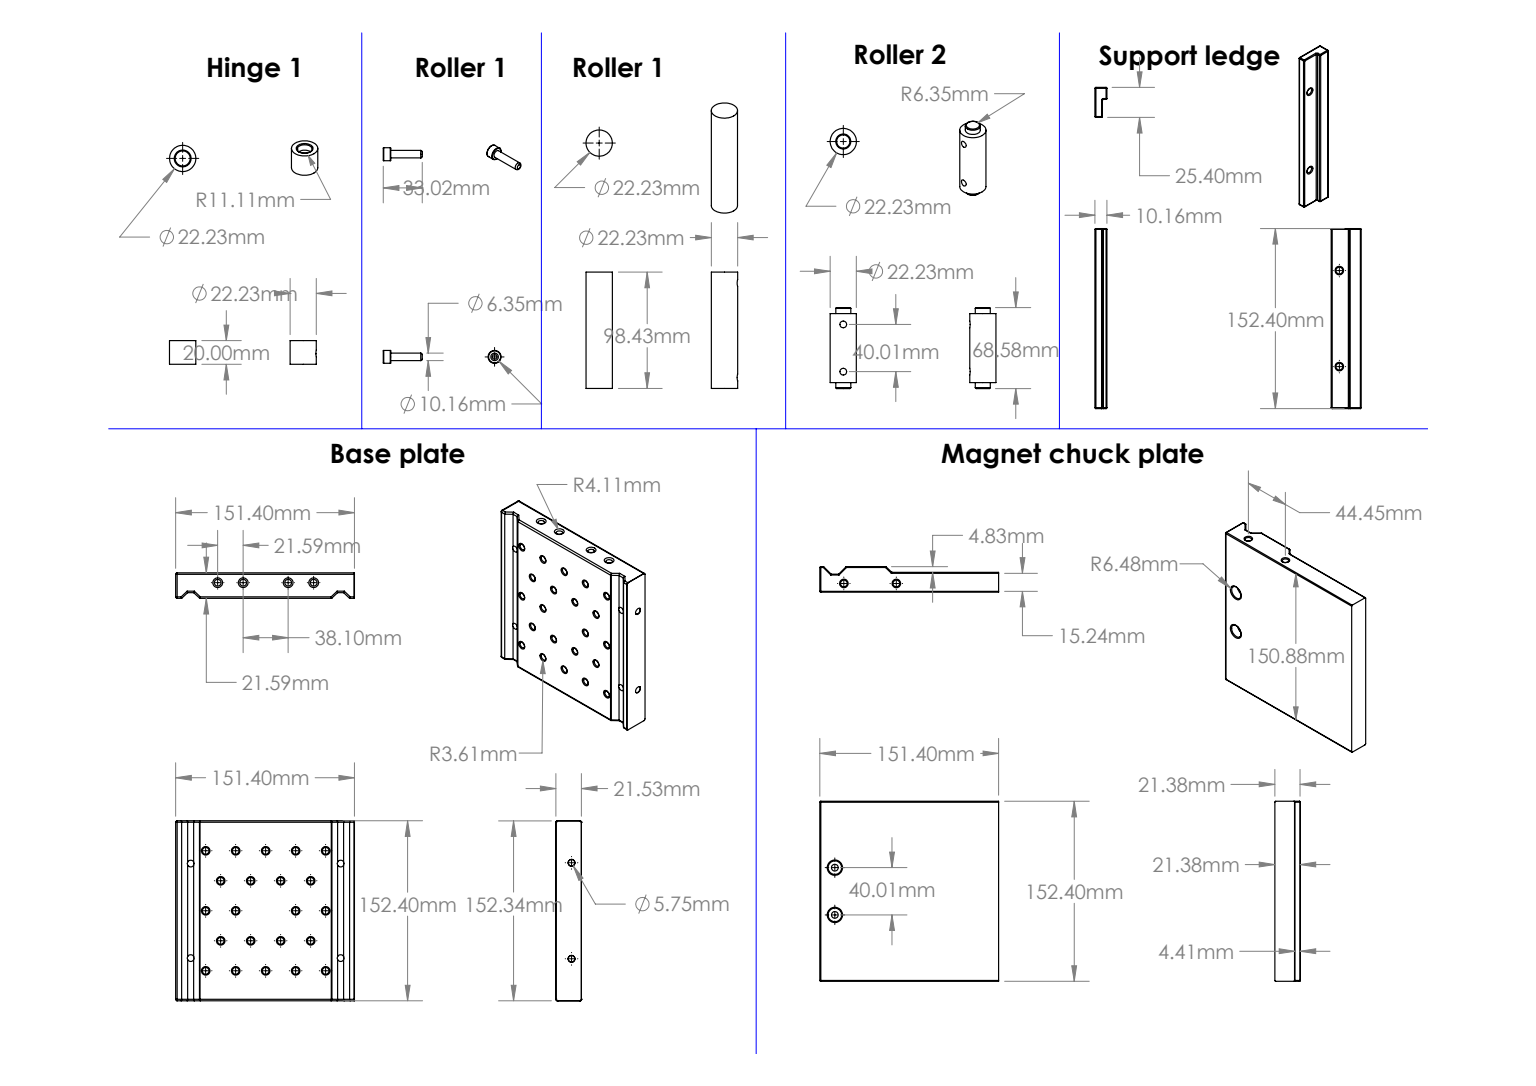
ISO-10303-21;
HEADER;
FILE_DESCRIPTION (('STEP AP214'),
    '1' );
FILE_NAME ('Hinge 1.step',
    '2026-10-26T17:37:43',
    ( '' ),
    ( '' ),
    'SwSTEP 2.0',
    'SolidWorks 2024',
    '' );
FILE_SCHEMA (( 'AUTOMOTIVE_DESIGN' ));
ENDSEC;

DATA;
#21=ORIENTED_EDGE ( 'NONE', *, *, #16592, .T. ) ;
#24=ORIENTED_EDGE ( 'NONE', *, *, #21540, .F. ) ;
#151=FACE_OUTER_BOUND ( 'NONE', #1516, .T. ) ;
#182=EDGE_CURVE ( 'NONE', #17917, #2186, #21094, .T. ) ;
#200=CIRCLE ( 'NONE', #6578, 0.7619999999999294005 ) ;
#366=CARTESIAN_POINT ( 'NONE',  ( 14.03509158661000100, -3662.022285901000032, 2257.672186979000344 ) ) ;
#368=DIRECTION ( 'NONE',  ( 0.000000000000000000, 0.000000000000000000, -1.000000000000000000 ) ) ;
#412=ORIENTED_EDGE ( 'NONE', *, *, #21540, .T. ) ;
#442=ORIENTED_EDGE ( 'NONE', *, *, #1926, .T. ) ;
#531=EDGE_CURVE ( 'NONE', #3180, #17789, #10470, .T. ) ;
#534=CARTESIAN_POINT ( 'NONE',  ( 15.54479972196000048, -3659.504990611520043, 2257.962943248000101 ) ) ;
#662=CIRCLE ( 'NONE', #16384, 11.11250000000000071 ) ;
#678=DIRECTION ( 'NONE',  ( 0.000000000000000000, 0.000000000000000000, -1.000000000000000000 ) ) ;
#714=ORIENTED_EDGE ( 'NONE', *, *, #9491, .T. ) ;
#740=EDGE_CURVE ( 'NONE', #9155, #17917, #6159, .T. ) ;
#785=PRODUCT ( 'Hinge 1', 'Hinge 1', '', ( #12191 ) ) ;
#806=ORIENTED_EDGE ( 'NONE', *, *, #17445, .T. ) ;
#1019=AXIS2_PLACEMENT_3D ( 'NONE', #14450, #2022, #21597 ) ;
#1040=ADVANCED_FACE ( 'NONE', ( #13493 ), #11393, .F. ) ;
#1091=ORIENTED_EDGE ( 'NONE', *, *, #12878, .T. ) ;
#1121=FACE_OUTER_BOUND ( 'NONE', #15842, .T. ) ;
#1168=TOROIDAL_SURFACE ( 'NONE', #14289, 7.112000000000000099, 0.7620000000000000107 ) ;
#1175=ORIENTED_EDGE ( 'NONE', *, *, #1982, .F. ) ;
#1239=AXIS2_PLACEMENT_3D ( 'NONE', #15381, #9530, #20423 ) ;
#1258=CARTESIAN_POINT ( 'NONE',  ( 12.70000020906999971, -3662.349800009999854, 2257.592639999999847 ) ) ;
#1275=PRODUCT_DEFINITION_CONTEXT ( 'detailed design', #14590, 'design' ) ;
#1366=EDGE_CURVE ( 'NONE', #17007, #3180, #17690, .T. ) ;
#1368=DIRECTION ( 'NONE',  ( 0.000000000000000000, -1.000000000000000000, 0.000000000000000000 ) ) ;
#1370=ORIENTED_EDGE ( 'NONE', *, *, #16592, .F. ) ;
#1382=CARTESIAN_POINT ( 'NONE',  ( 12.42421805959000025, -3662.340875907999816, 2257.594929573999707 ) ) ;
#1445=ORIENTED_EDGE ( 'NONE', *, *, #1366, .F. ) ;
#1489=CARTESIAN_POINT ( 'NONE',  ( 9.970475488813999476, -3658.687501247999990, 2257.932973791000222 ) ) ;
#1490=CARTESIAN_POINT ( 'NONE',  ( 11.12257588577000078, -3661.878010978000020, 2257.704312134999782 ) ) ;
#1516=EDGE_LOOP ( 'NONE', ( #13022, #20332, #9666, #3962 ) ) ;
#1545=AXIS2_PLACEMENT_3D ( 'NONE', #16930, #6293, #20459 ) ;
#1549=AXIS2_PLACEMENT_3D ( 'NONE', #16667, #9524, #18765 ) ;
#1593=VERTEX_POINT ( 'NONE', #21921 ) ;
#1607=CARTESIAN_POINT ( 'NONE',  ( 9.855200508358999301, -3659.413078923999819, 2257.962940201000038 ) ) ;
#1611=CARTESIAN_POINT ( 'NONE',  ( 12.69999999999999929, -3649.471999999999753, 2262.355140000000119 ) ) ;
#1732=CARTESIAN_POINT ( 'NONE',  ( 12.69999999999999929, -3655.060000000000400, 2268.705139999999574 ) ) ;
#1803=EDGE_LOOP ( 'NONE', ( #3126, #6623 ) ) ;
#1851=CARTESIAN_POINT ( 'NONE',  ( 10.49453184711000020, -3657.700682589000280, 2257.813182895999944 ) ) ;
#1876=DIRECTION ( 'NONE',  ( 0.000000000000000000, -1.000000000000000000, 0.000000000000000000 ) ) ;
#1926=EDGE_CURVE ( 'NONE', #5052, #15577, #13332, .T. ) ;
#1982=EDGE_CURVE ( 'NONE', #2186, #17917, #3455, .T. ) ;
#1998=DIRECTION ( 'NONE',  ( 0.000000000000000000, 0.000000000000000000, 1.000000000000000000 ) ) ;
#2016=PLANE ( 'NONE',  #20971 ) ;
#2022=DIRECTION ( 'NONE',  ( 0.000000000000000000, 1.000000000000000000, 0.000000000000000000 ) ) ;
#2056=VECTOR ( 'NONE', #21267, 1000.000000000000000 ) ;
#2132=CARTESIAN_POINT ( 'NONE',  ( 15.42948858069999929, -3660.322618741000042, 2257.932964559000084 ) ) ;
#2179=ORIENTED_EDGE ( 'NONE', *, *, #9491, .F. ) ;
#2186=VERTEX_POINT ( 'NONE', #13680 ) ;
#2241=ORIENTED_EDGE ( 'NONE', *, *, #182, .T. ) ;
#2257=( GEOMETRIC_REPRESENTATION_CONTEXT ( 3 ) GLOBAL_UNCERTAINTY_ASSIGNED_CONTEXT ( ( #16741 ) ) GLOBAL_UNIT_ASSIGNED_CONTEXT ( ( #21126, #3419, #23094 ) ) REPRESENTATION_CONTEXT ( 'NONE', 'WORKASPACE' ) );
#2282=DIRECTION ( 'NONE',  ( -1.000000000000000000, -0.000000000000000000, -0.000000000000000000 ) ) ;
#2451=CARTESIAN_POINT ( 'NONE',  ( 12.69999999999999929, -3655.060000000000400, 2262.355140000000119 ) ) ;
#2490=LINE ( 'NONE', #22263, #21072 ) ;
#2547=AXIS2_PLACEMENT_3D ( 'NONE', #19457, #3285, #21103 ) ;
#2606=CARTESIAN_POINT ( 'NONE',  ( 0.000000000000000000, 0.000000000000000000, 0.000000000000000000 ) ) ;
#2739=CARTESIAN_POINT ( 'NONE',  ( 12.69999999999999929, -3655.060000000000400, 2262.355140000000119 ) ) ;
#2769=DIRECTION ( 'NONE',  ( 0.000000000000000000, -1.000000000000000000, 0.000000000000000000 ) ) ;
#2788=CARTESIAN_POINT ( 'NONE',  ( 12.69999999999999929, -3656.660200000000259, 2257.592639999999847 ) ) ;
#2865=DIRECTION ( 'NONE',  ( 1.000000000000000000, 0.000000000000000000, 0.000000000000000000 ) ) ;
#2910=CARTESIAN_POINT ( 'NONE',  ( 9.855200508393229697, -3659.504999998446692, 2257.962940200992307 ) ) ;
#3080=ORIENTED_EDGE ( 'NONE', *, *, #3865, .F. ) ;
#3126=ORIENTED_EDGE ( 'NONE', *, *, #15553, .T. ) ;
#3140=CARTESIAN_POINT ( 'NONE',  ( 14.03517516284999900, -3656.987758144000054, 2257.672197071000028 ) ) ;
#3156=EDGE_LOOP ( 'NONE', ( #12594, #412 ) ) ;
#3180=VERTEX_POINT ( 'NONE', #6414 ) ;
#3206=CIRCLE ( 'NONE', #5096, 11.11250000000000071 ) ;
#3208=LINE ( 'NONE', #13881, #2056 ) ;
#3257=CARTESIAN_POINT ( 'NONE',  ( 12.15081356636999921, -3656.709137308999743, 2257.605105499000274 ) ) ;
#3258=CARTESIAN_POINT ( 'NONE',  ( 9.855200958505918152, -3659.596994900638038, 2257.962940081783472 ) ) ;
#3285=DIRECTION ( 'NONE',  ( 0.000000000000000000, -1.000000000000000000, 0.000000000000000000 ) ) ;
#3316=VERTEX_POINT ( 'NONE', #3346 ) ;
#3346=CARTESIAN_POINT ( 'NONE',  ( 12.69999999999999929, -3655.060000000000400, 2275.055139999999483 ) ) ;
#3419=( NAMED_UNIT ( * ) PLANE_ANGLE_UNIT ( ) SI_UNIT ( $, .RADIAN. ) );
#3450=AXIS2_PLACEMENT_3D ( 'NONE', #4410, #9682, #6296 ) ;
#3455=CIRCLE ( 'NONE', #8332, 6.349999999999855760 ) ;
#3630=CARTESIAN_POINT ( 'NONE',  ( 12.69999999999999929, -3648.710000000000036, 2268.705139999999574 ) ) ;
#3646=CARTESIAN_POINT ( 'NONE',  ( 12.79204376678999999, -3662.349799990000065, 2257.592639999999847 ) ) ;
#3651=CARTESIAN_POINT ( 'NONE',  ( 12.69999999999999929, -3655.060000000000400, 2268.705139999999574 ) ) ;
#3691=ADVANCED_FACE ( 'NONE', ( #151 ), #7297, .F. ) ;
#3753=DIRECTION ( 'NONE',  ( 1.000000000000000000, 0.000000000000000000, -1.224646799147353207E-16 ) ) ;
#3815=DIRECTION ( 'NONE',  ( 0.000000000000000000, 0.000000000000000000, -1.000000000000000000 ) ) ;
#3865=EDGE_CURVE ( 'NONE', #3889, #15577, #4425, .T. ) ;
#3889=VERTEX_POINT ( 'NONE', #14792 ) ;
#3962=ORIENTED_EDGE ( 'NONE', *, *, #182, .F. ) ;
#4078=ORIENTED_EDGE ( 'NONE', *, *, #13162, .T. ) ;
#4242=CIRCLE ( 'NONE', #4993, 7.111999999999785160 ) ;
#4284=CARTESIAN_POINT ( 'NONE',  ( 12.69999999999999929, -3648.710000000000036, 2268.705139999999574 ) ) ;
#4338=TOROIDAL_SURFACE ( 'NONE', #11437, 7.112000000000000099, 0.7620000000000000107 ) ;
#4410=CARTESIAN_POINT ( 'NONE',  ( 12.69999999999999929, -3659.504999999999654, 2272.030000000000200 ) ) ;
#4425=B_SPLINE_CURVE_WITH_KNOTS ( 'NONE', 3,
 ( #5899, #13036, #11267, #18414 ),
 .UNSPECIFIED., .F., .F.,
 ( 4, 4 ),
 ( 0.000000000000000000, 3.168591426078622932E-06 ),
 .UNSPECIFIED. ) ;
#4428=DIRECTION ( 'NONE',  ( 0.000000000000000000, -1.000000000000000000, 0.000000000000000000 ) ) ;
#4511=EDGE_CURVE ( 'NONE', #8413, #3889, #6339, .T. ) ;
#4544=CARTESIAN_POINT ( 'NONE',  ( 14.27729191008000065, -3657.131900051000230, 2257.704292951999832 ) ) ;
#4585=CIRCLE ( 'NONE', #14342, 11.11250000000000071 ) ;
#4649=CIRCLE ( 'NONE', #13636, 2.844799999999999773 ) ;
#4722=CARTESIAN_POINT ( 'NONE',  ( 12.70000000000000107, -3668.712499999999636, 2279.817639999999756 ) ) ;
#4746=CARTESIAN_POINT ( 'NONE',  ( 12.69999999999999929, -3668.712499999999636, 2268.705139999999574 ) ) ;
#4883=LINE ( 'NONE', #17411, #16568 ) ;
#4898=CARTESIAN_POINT ( 'NONE',  ( 10.32639513556999944, -3661.081539619000068, 2257.848705702999723 ) ) ;
#4936=DIRECTION ( 'NONE',  ( 0.000000000000000000, -1.000000000000000000, 0.000000000000000000 ) ) ;
#4993=AXIS2_PLACEMENT_3D ( 'NONE', #3630, #1876, #1998 ) ;
#5021=CARTESIAN_POINT ( 'NONE',  ( 9.855200508358999301, -3659.504986005999854, 2257.962940201000038 ) ) ;
#5032=ORIENTED_EDGE ( 'NONE', *, *, #12878, .F. ) ;
#5052=VERTEX_POINT ( 'NONE', #22901 ) ;
#5096=AXIS2_PLACEMENT_3D ( 'NONE', #8757, #14264, #10622 ) ;
#5144=CARTESIAN_POINT ( 'NONE',  ( 10.18227454630999951, -3660.839269783999953, 2257.881334183000035 ) ) ;
#5186=VERTEX_POINT ( 'NONE', #16684 ) ;
#5254=CARTESIAN_POINT ( 'NONE',  ( 12.69999999999999929, -3659.504999999999654, 2272.030000000000200 ) ) ;
#5439=EDGE_LOOP ( 'NONE', ( #1091, #9150 ) ) ;
#5541=CARTESIAN_POINT ( 'NONE',  ( 15.21766708706000060, -3660.839381832000072, 2257.881320499000140 ) ) ;
#5605=DIRECTION ( 'NONE',  ( 0.000000000000000000, 0.000000000000000000, -1.000000000000000000 ) ) ;
#5611=AXIS2_PLACEMENT_3D ( 'NONE', #2606, #9751, #7545 ) ;
#5680=CIRCLE ( 'NONE', #7178, 6.349999999999855760 ) ;
#5770=CARTESIAN_POINT ( 'NONE',  ( 13.24911585008999815, -3662.300876935000360, 2257.605101898000157 ) ) ;
#5801=( LENGTH_UNIT ( ) NAMED_UNIT ( * ) SI_UNIT ( .MILLI., .METRE. ) );
#5815=EDGE_CURVE ( 'NONE', #17789, #8413, #6051, .T. ) ;
#5838=MANIFOLD_SOLID_BREP ( 'SOLID2-15[1]', #16587 ) ;
#5899=CARTESIAN_POINT ( 'NONE',  ( 9.855200508358999301, -3659.504986005999854, 2257.962940201000038 ) ) ;
#5928=ORIENTED_EDGE ( 'NONE', *, *, #13887, .F. ) ;
#5991=EDGE_CURVE ( 'NONE', #6867, #3180, #10524, .T. ) ;
#6027=( NAMED_UNIT ( * ) PLANE_ANGLE_UNIT ( ) SI_UNIT ( $, .RADIAN. ) );
#6028=FACE_OUTER_BOUND ( 'NONE', #11655, .T. ) ;
#6051=B_SPLINE_CURVE_WITH_KNOTS ( 'NONE', 3,
 ( #6557, #10051, #12047, #17081, #6678, #11814, #19203, #6786, #13816, #13927, #13457, #4544, #3140, #22584, #11687, #18844, #21077, #8074, #2788 ),
 .UNSPECIFIED., .F., .F.,
 ( 4, 1, 1, 1, 1, 1, 1, 1, 1, 1, 1, 1, 1, 1, 1, 1, 4 ),
 ( 0.000000000000000000, 0.06250000000000000000, 0.1250000000000000000, 0.1875000000000000000, 0.2500000000000000000, 0.3125000000000000000, 0.3750000000000000000, 0.4375000000000000000, 0.5000000000000000000, 0.5625000000000000000, 0.6250000000000000000, 0.6875000000000000000, 0.7500000000000000000, 0.8125000000000000000, 0.8750000000000000000, 0.9375000000000000000, 1.000000000000000000 ),
 .UNSPECIFIED. ) ;
#6159=LINE ( 'NONE', #2739, #19136 ) ;
#6179=ORIENTED_EDGE ( 'NONE', *, *, #13727, .T. ) ;
#6188=DIRECTION ( 'NONE',  ( 0.000000000000000000, 0.000000000000000000, -1.000000000000000000 ) ) ;
#6293=DIRECTION ( 'NONE',  ( 0.000000000000000000, 1.000000000000000000, 0.000000000000000000 ) ) ;
#6296=DIRECTION ( 'NONE',  ( -1.000000000000000000, 0.000000000000000000, 0.000000000000000000 ) ) ;
#6339=B_SPLINE_CURVE_WITH_KNOTS ( 'NONE', 3,
 ( #21423, #7025, #12164, #3257, #21542, #13924, #10403, #17543, #19785, #19544, #1851, #6784, #22925, #19430, #1489, #10632, #14393, #1607, #5021 ),
 .UNSPECIFIED., .F., .F.,
 ( 4, 1, 1, 1, 1, 1, 1, 1, 1, 1, 1, 1, 1, 1, 1, 1, 4 ),
 ( 0.000000000000000000, 0.06250000000000000000, 0.1250000000000000000, 0.1875000000000000000, 0.2500000000000000000, 0.3125000000000000000, 0.3750000000000000000, 0.4375000000000000000, 0.5000000000000000000, 0.5625000000000000000, 0.6250000000000000000, 0.6875000000000000000, 0.7500000000000000000, 0.8125000000000000000, 0.8750000000000000000, 0.9375000000000000000, 1.000000000000000000 ),
 .UNSPECIFIED. ) ;
#6414=CARTESIAN_POINT ( 'NONE',  ( 15.54479972192533488, -3659.504999998566745, 2257.962943247991007 ) ) ;
#6557=CARTESIAN_POINT ( 'NONE',  ( 15.54479972196000048, -3659.504985917999875, 2257.962943248000101 ) ) ;
#6578=AXIS2_PLACEMENT_3D ( 'NONE', #19825, #3753, #368 ) ;
#6608=CARTESIAN_POINT ( 'NONE',  ( 12.69999999999999929, -3648.710000000000036, 2268.705139999999574 ) ) ;
#6623=ORIENTED_EDGE ( 'NONE', *, *, #15321, .T. ) ;
#6676=CARTESIAN_POINT ( 'NONE',  ( 9.864080040025308804, -3659.780148078739330, 2257.960588549625299 ) ) ;
#6678=CARTESIAN_POINT ( 'NONE',  ( 15.42952381853999988, -3658.687498958000106, 2257.932973515999947 ) ) ;
#6721=CARTESIAN_POINT ( 'NONE',  ( 12.69999999999999929, -3648.710000000000036, 2257.592639999999847 ) ) ;
#6753=DIRECTION ( 'NONE',  ( 0.000000000000000000, -1.000000000000000000, 0.000000000000000000 ) ) ;
#6784=CARTESIAN_POINT ( 'NONE',  ( 10.32641459757000035, -3657.928429337000125, 2257.848701351999807 ) ) ;
#6786=CARTESIAN_POINT ( 'NONE',  ( 15.07358448401000217, -3657.928427944000305, 2257.848701151000114 ) ) ;
#6867=VERTEX_POINT ( 'NONE', #20304 ) ;
#6920=FACE_OUTER_BOUND ( 'NONE', #3156, .T. ) ;
#6934=CARTESIAN_POINT ( 'NONE',  ( 12.69999999999999929, -3648.710000000000036, 2261.593139999999948 ) ) ;
#6985=SHAPE_REPRESENTATION ( 'Hinge 1', ( #5611 ), #14218 ) ;
#7025=CARTESIAN_POINT ( 'NONE',  ( 12.60791899384999937, -3656.660200000000259, 2257.592639999999847 ) ) ;
#7027=VERTEX_POINT ( 'NONE', #6934 ) ;
#7038=VECTOR ( 'NONE', #16603, 1000.000000000000000 ) ;
#7178=AXIS2_PLACEMENT_3D ( 'NONE', #1732, #16253, #5605 ) ;
#7245=DIRECTION ( 'NONE',  ( 0.000000000000000000, -1.000000000000000000, 0.000000000000000000 ) ) ;
#7297=CYLINDRICAL_SURFACE ( 'NONE', #1019, 6.349999999999855760 ) ;
#7358=AXIS2_PLACEMENT_3D ( 'NONE', #4284, #18576, #7914 ) ;
#7425=VERTEX_POINT ( 'NONE', #4722 ) ;
#7459=ADVANCED_FACE ( 'NONE', ( #10098 ), #12330, .T. ) ;
#7510=CARTESIAN_POINT ( 'NONE',  ( 15.49598722424000030, -3660.053501552999933, 2257.950090894999903 ) ) ;
#7540=CIRCLE ( 'NONE', #1545, 6.349999999999855760 ) ;
#7545=DIRECTION ( 'NONE',  ( 1.000000000000000000, 0.000000000000000000, 0.000000000000000000 ) ) ;
#7637=ADVANCED_FACE ( 'NONE', ( #16418 ), #2016, .T. ) ;
#7677=CARTESIAN_POINT ( 'NONE',  ( 15.54479972196000048, -3659.504985917999875, 2257.962943248000101 ) ) ;
#7732=SHAPE_DEFINITION_REPRESENTATION ( #20441, #6985 ) ;
#7837=UNCERTAINTY_MEASURE_WITH_UNIT (LENGTH_MEASURE( 1.000000000000000082E-05 ), #5801, 'distance_accuracy_value', 'NONE');
#7914=DIRECTION ( 'NONE',  ( 0.000000000000000000, 0.000000000000000000, 1.000000000000000000 ) ) ;
#7943=CARTESIAN_POINT ( 'NONE',  ( 12.69999999999999929, -3648.710000000000036, 2268.705139999999574 ) ) ;
#7944=CIRCLE ( 'NONE', #21045, 11.11250000000000071 ) ;
#7948=CARTESIAN_POINT ( 'NONE',  ( 9.855199999999999960, -3659.504999999999654, 2272.030000000000200 ) ) ;
#8065=FACE_OUTER_BOUND ( 'NONE', #11000, .T. ) ;
#8074=CARTESIAN_POINT ( 'NONE',  ( 12.79208108087000006, -3656.660200000000259, 2257.592639999999847 ) ) ;
#8172=CARTESIAN_POINT ( 'NONE',  ( 12.69999999999999929, -3649.471999999999753, 2268.705139999999574 ) ) ;
#8180=DIRECTION ( 'NONE',  ( -1.000000000000000000, 0.000000000000000000, 0.000000000000000000 ) ) ;
#8223=CARTESIAN_POINT ( 'NONE',  ( 12.69999999999999929, -3649.471999999999753, 2268.705139999999574 ) ) ;
#8231=ORIENTED_EDGE ( 'NONE', *, *, #1926, .F. ) ;
#8248=PRODUCT_DEFINITION_FORMATION_WITH_SPECIFIED_SOURCE ( 'ANY', '', #785, .NOT_KNOWN. ) ;
#8305=CARTESIAN_POINT ( 'NONE',  ( 11.61844525849999954, -3662.141125287999785, 2257.644379465999918 ) ) ;
#8309=ORIENTED_EDGE ( 'NONE', *, *, #10357, .F. ) ;
#8332=AXIS2_PLACEMENT_3D ( 'NONE', #20479, #4428, #18374 ) ;
#8413=VERTEX_POINT ( 'NONE', #13272 ) ;
#8462=CIRCLE ( 'NONE', #13691, 2.844799999999999773 ) ;
#8560=VERTEX_POINT ( 'NONE', #6721 ) ;
#8757=CARTESIAN_POINT ( 'NONE',  ( 12.69999999999999929, -3668.712499999999636, 2268.705139999999574 ) ) ;
#8831=ORIENTED_EDGE ( 'NONE', *, *, #5991, .T. ) ;
#8888=DIRECTION ( 'NONE',  ( 1.000000000000000000, 0.000000000000000000, 0.000000000000000000 ) ) ;
#8955=ADVANCED_FACE ( 'NONE', ( #6920 ), #13834, .T. ) ;
#9150=ORIENTED_EDGE ( 'NONE', *, *, #10357, .T. ) ;
#9155=VERTEX_POINT ( 'NONE', #2451 ) ;
#9188=ORIENTED_EDGE ( 'NONE', *, *, #5815, .F. ) ;
#9318=CARTESIAN_POINT ( 'NONE',  ( 12.69999999999999929, -3649.471999999999753, 2261.593139999999948 ) ) ;
#9491=EDGE_CURVE ( 'NONE', #8560, #1593, #662, .T. ) ;
#9524=DIRECTION ( 'NONE',  ( 0.000000000000000000, 0.000000000000000000, 1.000000000000000000 ) ) ;
#9530=DIRECTION ( 'NONE',  ( 0.000000000000000000, 1.000000000000000000, 0.000000000000000000 ) ) ;
#9559=DIRECTION ( 'NONE',  ( 0.000000000000000000, -1.000000000000000000, 0.000000000000000000 ) ) ;
#9666=ORIENTED_EDGE ( 'NONE', *, *, #17249, .T. ) ;
#9682=DIRECTION ( 'NONE',  ( 0.000000000000000000, 0.000000000000000000, -1.000000000000000000 ) ) ;
#9751=DIRECTION ( 'NONE',  ( 0.000000000000000000, 0.000000000000000000, 1.000000000000000000 ) ) ;
#9857=ORIENTED_EDGE ( 'NONE', *, *, #17445, .F. ) ;
#9865=ORIENTED_EDGE ( 'NONE', *, *, #16471, .T. ) ;
#9923=ADVANCED_FACE ( 'NONE', ( #16878, #11494 ), #18644, .F. ) ;
#10049=CARTESIAN_POINT ( 'NONE',  ( 9.904004635912999177, -3660.053455317999578, 2257.950092655999924 ) ) ;
#10051=CARTESIAN_POINT ( 'NONE',  ( 15.54479972196000048, -3659.413078500999745, 2257.962943248000101 ) ) ;
#10098=FACE_OUTER_BOUND ( 'NONE', #18381, .T. ) ;
#10239=EDGE_CURVE ( 'NONE', #15577, #17007, #22466, .T. ) ;
#10285=CARTESIAN_POINT ( 'NONE',  ( 9.970491213060000746, -3660.322548418000224, 2257.932969814999979 ) ) ;
#10357=EDGE_CURVE ( 'NONE', #6867, #5052, #8462, .T. ) ;
#10403=CARTESIAN_POINT ( 'NONE',  ( 11.36482343738000012, -3656.987758866999684, 2257.672197237000091 ) ) ;
#10470=B_SPLINE_CURVE_WITH_KNOTS ( 'NONE', 3,
 ( #21639, #16581, #534, #7677 ),
 .UNSPECIFIED., .F., .F.,
 ( 4, 4 ),
 ( 0.9999968116805088014, 1.000000000000000000 ),
 .UNSPECIFIED. ) ;
#10524=LINE ( 'NONE', #20019, #7038 ) ;
#10546=CARTESIAN_POINT ( 'NONE',  ( 12.69999999999999929, -3668.712499999999636, 2268.705139999999574 ) ) ;
#10550=AXIS2_PLACEMENT_3D ( 'NONE', #9318, #2282, #13165 ) ;
#10622=DIRECTION ( 'NONE',  ( 1.000000000000000000, 0.000000000000000000, 3.996303350731721563E-14 ) ) ;
#10631=CARTESIAN_POINT ( 'NONE',  ( 12.69999999999999929, -3648.710000000000036, 2268.705139999999574 ) ) ;
#10632=CARTESIAN_POINT ( 'NONE',  ( 9.903987878842999137, -3658.956623412000226, 2257.950097015999745 ) ) ;
#10796=CARTESIAN_POINT ( 'NONE',  ( 14.71507054554999883, -3661.519743953000216, 2257.776232814999730 ) ) ;
#10854=CARTESIAN_POINT ( 'NONE',  ( 12.69999999999999929, -3659.504999999999654, 2272.030000000000200 ) ) ;
#10911=CARTESIAN_POINT ( 'NONE',  ( 14.50480255619999959, -3661.710066511000150, 2257.739429448999999 ) ) ;
#11000=EDGE_LOOP ( 'NONE', ( #8309, #8831, #1445, #13214, #8231 ) ) ;
#11003=ORIENTED_EDGE ( 'NONE', *, *, #3865, .T. ) ;
#11267=CARTESIAN_POINT ( 'NONE',  ( 9.855200508370408841, -3659.504995334291834, 2257.962940200996854 ) ) ;
#11341=DIRECTION ( 'NONE',  ( 0.000000000000000000, 0.000000000000000000, -1.000000000000000000 ) ) ;
#11393=PLANE ( 'NONE',  #1549 ) ;
#11433=FACE_OUTER_BOUND ( 'NONE', #11545, .T. ) ;
#11437=AXIS2_PLACEMENT_3D ( 'NONE', #8172, #20695, #6188 ) ;
#11494=FACE_OUTER_BOUND ( 'NONE', #16090, .T. ) ;
#11501=ORIENTED_EDGE ( 'NONE', *, *, #740, .T. ) ;
#11520=CARTESIAN_POINT ( 'NONE',  ( 12.70000020906999971, -3662.349800009999854, 2257.592639999999847 ) ) ;
#11545=EDGE_LOOP ( 'NONE', ( #16831, #5032, #442, #3080, #16616, #9188, #12453 ) ) ;
#11655=EDGE_LOOP ( 'NONE', ( #15097, #11501, #1175, #17613 ) ) ;
#11673=DIRECTION ( 'NONE',  ( 0.000000000000000000, 0.000000000000000000, -1.000000000000000000 ) ) ;
#11687=CARTESIAN_POINT ( 'NONE',  ( 13.51849986531999903, -3656.775770755999929, 2257.621751478000078 ) ) ;
#11814=CARTESIAN_POINT ( 'NONE',  ( 15.33662675678000120, -3658.424664496000332, 2257.909780506000061 ) ) ;
#11977=DIRECTION ( 'NONE',  ( 0.000000000000000000, -1.000000000000000000, 0.000000000000000000 ) ) ;
#12047=CARTESIAN_POINT ( 'NONE',  ( 15.53593155406000115, -3659.229969269999856, 2257.960590233999937 ) ) ;
#12084=DIRECTION ( 'NONE',  ( 0.000000000000000000, 0.000000000000000000, 1.000000000000000000 ) ) ;
#12164=CARTESIAN_POINT ( 'NONE',  ( 12.42449270472999956, -3656.669101290000071, 2257.594923725999706 ) ) ;
#12191=PRODUCT_CONTEXT ( 'NONE', #22030, 'mechanical' ) ;
#12310=DIRECTION ( 'NONE',  ( 0.000000000000000000, 0.000000000000000000, -1.000000000000000000 ) ) ;
#12330=CYLINDRICAL_SURFACE ( 'NONE', #13328, 11.11249999999985860 ) ;
#12434=ADVANCED_FACE ( 'NONE', ( #17179 ), #22217, .T. ) ;
#12440=CARTESIAN_POINT ( 'NONE',  ( 15.07352087697999998, -3661.081667652999840, 2257.848687205999795 ) ) ;
#12446=DIRECTION ( 'NONE',  ( -0.000000000000000000, 1.000000000000000000, 0.000000000000000000 ) ) ;
#12453=ORIENTED_EDGE ( 'NONE', *, *, #531, .F. ) ;
#12557=CARTESIAN_POINT ( 'NONE',  ( 14.27720943205999937, -3661.878154638000524, 2257.704281108000032 ) ) ;
#12594=ORIENTED_EDGE ( 'NONE', *, *, #14152, .T. ) ;
#12628=EDGE_LOOP ( 'NONE', ( #15248, #4078, #18631, #5928, #21559, #19497, #17745, #1370 ) ) ;
#12743=LINE ( 'NONE', #16031, #18421 ) ;
#12878=EDGE_CURVE ( 'NONE', #5052, #6867, #4649, .T. ) ;
#12900=CARTESIAN_POINT ( 'NONE',  ( 14.90539642439000012, -3661.309404879999875, 2257.813168336999752 ) ) ;
#12931=ORIENTED_EDGE ( 'NONE', *, *, #15951, .F. ) ;
#13022=ORIENTED_EDGE ( 'NONE', *, *, #740, .F. ) ;
#13036=CARTESIAN_POINT ( 'NONE',  ( 9.855200508358999301, -3659.504990670146526, 2257.962940201000038 ) ) ;
#13160=CYLINDRICAL_SURFACE ( 'NONE', #1239, 6.349999999999855760 ) ;
#13162=EDGE_CURVE ( 'NONE', #1593, #7425, #3208, .T. ) ;
#13165=DIRECTION ( 'NONE',  ( 0.000000000000000000, 0.000000000000000000, 1.000000000000000000 ) ) ;
#13214=ORIENTED_EDGE ( 'NONE', *, *, #10239, .F. ) ;
#13272=CARTESIAN_POINT ( 'NONE',  ( 12.69999999999999929, -3656.660200000000259, 2257.592639999999847 ) ) ;
#13328=AXIS2_PLACEMENT_3D ( 'NONE', #6608, #11977, #22511 ) ;
#13332=LINE ( 'NONE', #7948, #13935 ) ;
#13333=ORIENTED_EDGE ( 'NONE', *, *, #13162, .F. ) ;
#13457=CARTESIAN_POINT ( 'NONE',  ( 14.50488223892000050, -3657.299998513999981, 2257.739442581999810 ) ) ;
#13493=FACE_OUTER_BOUND ( 'NONE', #5439, .T. ) ;
#13577=CARTESIAN_POINT ( 'NONE',  ( 11.36465921565999970, -3662.022152739999456, 2257.672217410000030 ) ) ;
#13636=AXIS2_PLACEMENT_3D ( 'NONE', #10854, #3815, #2865 ) ;
#13680=CARTESIAN_POINT ( 'NONE',  ( 12.69999999999999929, -3649.471999999999753, 2275.055139999999483 ) ) ;
#13690=DIRECTION ( 'NONE',  ( 0.000000000000000000, 1.000000000000000000, 0.000000000000000000 ) ) ;
#13691=AXIS2_PLACEMENT_3D ( 'NONE', #5254, #19545, #8888 ) ;
#13727=EDGE_CURVE ( 'NONE', #2186, #19565, #200, .T. ) ;
#13816=CARTESIAN_POINT ( 'NONE',  ( 14.90546723228000126, -3657.700681481000174, 2257.813182709000102 ) ) ;
#13834=PLANE ( 'NONE',  #17110 ) ;
#13881=CARTESIAN_POINT ( 'NONE',  ( 12.70000000000000107, -3648.710000000000036, 2279.817639999999756 ) ) ;
#13887=EDGE_CURVE ( 'NONE', #17007, #5186, #4883, .T. ) ;
#13924=CARTESIAN_POINT ( 'NONE',  ( 11.61864837389999927, -3656.868790608999916, 2257.644359388999874 ) ) ;
#13925=CARTESIAN_POINT ( 'NONE',  ( 10.06338274650999942, -3660.585356121999666, 2257.909778189000008 ) ) ;
#13927=CARTESIAN_POINT ( 'NONE',  ( 14.71514678359000072, -3657.490332083999874, 2257.776246897999954 ) ) ;
#13930=AXIS2_PLACEMENT_3D ( 'NONE', #18609, #11341, #8180 ) ;
#13935=VECTOR ( 'NONE', #11673, 1000.000000000000000 ) ;
#14043=CARTESIAN_POINT ( 'NONE',  ( 12.60780787143999859, -3662.349800030000097, 2257.592639999999847 ) ) ;
#14152=EDGE_CURVE ( 'NONE', #5186, #7425, #4585, .T. ) ;
#14218=( GEOMETRIC_REPRESENTATION_CONTEXT ( 3 ) GLOBAL_UNCERTAINTY_ASSIGNED_CONTEXT ( ( #7837 ) ) GLOBAL_UNIT_ASSIGNED_CONTEXT ( ( #5801, #6027, #14815 ) ) REPRESENTATION_CONTEXT ( 'NONE', 'WORKASPACE' ) );
#14264=DIRECTION ( 'NONE',  ( 0.000000000000000000, -1.000000000000000000, 0.000000000000000000 ) ) ;
#14289=AXIS2_PLACEMENT_3D ( 'NONE', #22896, #6753, #15655 ) ;
#14342=AXIS2_PLACEMENT_3D ( 'NONE', #4746, #9559, #16704 ) ;
#14393=CARTESIAN_POINT ( 'NONE',  ( 9.864068217991999177, -3659.229970544000025, 2257.960591680000107 ) ) ;
#14437=AXIS2_PLACEMENT_3D ( 'NONE', #7943, #2769, #678 ) ;
#14450=CARTESIAN_POINT ( 'NONE',  ( 12.69999999999999929, -3655.060000000000400, 2268.705139999999574 ) ) ;
#14480=ADVANCED_FACE ( 'NONE', ( #6028 ), #13160, .F. ) ;
#14590=APPLICATION_CONTEXT ( 'configuration controlled 3d designs of mechanical parts and assemblies' ) ;
#14666=CARTESIAN_POINT ( 'NONE',  ( 15.54479926893309027, -3659.597001414151691, 2257.962943127797644 ) ) ;
#14792=CARTESIAN_POINT ( 'NONE',  ( 9.855200508358999301, -3659.504986005999854, 2257.962940201000038 ) ) ;
#14815=( NAMED_UNIT ( * ) SI_UNIT ( $, .STERADIAN. ) SOLID_ANGLE_UNIT ( ) );
#14965=ORIENTED_EDGE ( 'NONE', *, *, #13887, .T. ) ;
#15053=ORIENTED_EDGE ( 'NONE', *, *, #1982, .T. ) ;
#15097=ORIENTED_EDGE ( 'NONE', *, *, #15321, .F. ) ;
#15111=ADVANCED_FACE ( 'NONE', ( #8065 ), #20484, .F. ) ;
#15234=ADVANCED_BREP_SHAPE_REPRESENTATION ( '', ( #5838, #5611 ), #14218 ) ;
#15248=ORIENTED_EDGE ( 'NONE', *, *, #16471, .F. ) ;
#15277=DIRECTION ( 'NONE',  ( 0.000000000000000000, 1.000000000000000000, 0.000000000000000000 ) ) ;
#15321=EDGE_CURVE ( 'NONE', #9155, #3316, #5680, .T. ) ;
#15381=CARTESIAN_POINT ( 'NONE',  ( 12.69999999999999929, -3655.060000000000400, 2268.705139999999574 ) ) ;
#15449=CARTESIAN_POINT ( 'NONE',  ( 12.15052771711000013, -3662.300804947000415, 2257.605120077999800 ) ) ;
#15469=AXIS2_PLACEMENT_3D ( 'NONE', #8223, #4936, #12084 ) ;
#15503=ORIENTED_EDGE ( 'NONE', *, *, #13727, .F. ) ;
#15553=EDGE_CURVE ( 'NONE', #3316, #9155, #7540, .T. ) ;
#15577=VERTEX_POINT ( 'NONE', #22203 ) ;
#15655=DIRECTION ( 'NONE',  ( 0.000000000000000000, 0.000000000000000000, -1.000000000000000000 ) ) ;
#15687=ADVANCED_FACE ( 'NONE', ( #18929 ), #1168, .T. ) ;
#15811=EDGE_LOOP ( 'NONE', ( #22245, #806 ) ) ;
#15842=EDGE_LOOP ( 'NONE', ( #2241, #6179, #17843, #12931 ) ) ;
#15951=EDGE_CURVE ( 'NONE', #17917, #7027, #22131, .T. ) ;
#16031=CARTESIAN_POINT ( 'NONE',  ( 12.69999999999999929, -3648.710000000000036, 2257.592639999999847 ) ) ;
#16090=EDGE_LOOP ( 'NONE', ( #714, #9865 ) ) ;
#16188=CARTESIAN_POINT ( 'NONE',  ( 15.54479972192533488, -3659.504999998566745, 2257.962943247991007 ) ) ;
#16253=DIRECTION ( 'NONE',  ( 0.000000000000000000, 1.000000000000000000, 0.000000000000000000 ) ) ;
#16293=CARTESIAN_POINT ( 'NONE',  ( 12.70000000000000107, -3648.710000000000036, 2275.817139999999654 ) ) ;
#16384=AXIS2_PLACEMENT_3D ( 'NONE', #22288, #15277, #22402 ) ;
#16413=CARTESIAN_POINT ( 'NONE',  ( 12.70000020906999971, -3662.349800009999854, 2257.592639999999847 ) ) ;
#16418=FACE_OUTER_BOUND ( 'NONE', #1803, .T. ) ;
#16471=EDGE_CURVE ( 'NONE', #1593, #8560, #7944, .T. ) ;
#16526=CARTESIAN_POINT ( 'NONE',  ( 13.51841762737000074, -3662.234253382000134, 2257.621745511999961 ) ) ;
#16568=VECTOR ( 'NONE', #1368, 1000.000000000000000 ) ;
#16581=CARTESIAN_POINT ( 'NONE',  ( 15.54479972194844528, -3659.504995305038847, 2257.962943247996918 ) ) ;
#16587=CLOSED_SHELL ( 'NONE', ( #12434, #15111, #20108, #14480, #7637, #3691, #15687, #9923, #1040, #16719, #8955, #7459 ) ) ;
#16592=EDGE_CURVE ( 'NONE', #8560, #8413, #12743, .T. ) ;
#16603=DIRECTION ( 'NONE',  ( 0.000000000000000000, 0.000000000000000000, -1.000000000000000000 ) ) ;
#16616=ORIENTED_EDGE ( 'NONE', *, *, #4511, .F. ) ;
#16667=CARTESIAN_POINT ( 'NONE',  ( 12.69999999999999929, -3659.504999999999654, 2272.030000000000200 ) ) ;
#16684=CARTESIAN_POINT ( 'NONE',  ( 12.69999999999999929, -3668.712499999999636, 2257.592639999999847 ) ) ;
#16689=CIRCLE ( 'NONE', #7358, 7.111999999999785160 ) ;
#16704=DIRECTION ( 'NONE',  ( 1.000000000000000000, 0.000000000000000000, 3.996303350731721563E-14 ) ) ;
#16719=ADVANCED_FACE ( 'NONE', ( #11433 ), #22205, .F. ) ;
#16741=UNCERTAINTY_MEASURE_WITH_UNIT (LENGTH_MEASURE( 1.000000000000000082E-05 ), #21126, 'distance_accuracy_value', 'NONE');
#16831=ORIENTED_EDGE ( 'NONE', *, *, #5991, .F. ) ;
#16878=FACE_BOUND ( 'NONE', #15811, .T. ) ;
#16930=CARTESIAN_POINT ( 'NONE',  ( 12.69999999999999929, -3655.060000000000400, 2268.705139999999574 ) ) ;
#17007=VERTEX_POINT ( 'NONE', #11520 ) ;
#17081=CARTESIAN_POINT ( 'NONE',  ( 15.49601198374999989, -3658.956622429000163, 2257.950097350999840 ) ) ;
#17110=AXIS2_PLACEMENT_3D ( 'NONE', #10546, #21221, #12310 ) ;
#17179=FACE_OUTER_BOUND ( 'NONE', #12628, .T. ) ;
#17196=CARTESIAN_POINT ( 'NONE',  ( 10.49449033964999956, -3661.309265058999699, 2257.813191440000082 ) ) ;
#17249=EDGE_CURVE ( 'NONE', #3316, #2186, #2490, .T. ) ;
#17312=CARTESIAN_POINT ( 'NONE',  ( 11.88126810894999963, -3662.234158427000239, 2257.621768944999985 ) ) ;
#17411=CARTESIAN_POINT ( 'NONE',  ( 12.69999999999999929, -3648.710000000000036, 2257.592639999999847 ) ) ;
#17428=CARTESIAN_POINT ( 'NONE',  ( 10.89501796730999850, -3661.709918484999889, 2257.739459224999791 ) ) ;
#17445=EDGE_CURVE ( 'NONE', #19565, #7027, #4242, .T. ) ;
#17499=EDGE_LOOP ( 'NONE', ( #15503, #15053, #23117, #9857 ) ) ;
#17543=CARTESIAN_POINT ( 'NONE',  ( 11.12270644712000056, -3657.131901141000071, 2257.704293189000055 ) ) ;
#17613=ORIENTED_EDGE ( 'NONE', *, *, #17249, .F. ) ;
#17690=B_SPLINE_CURVE_WITH_KNOTS ( 'NONE', 3,
 ( #16413, #3646, #17936, #5770, #16526, #19824, #366, #12557, #10911, #10796, #12900, #12440, #5541, #18059, #2132, #7510, #19713, #14666, #16188 ),
 .UNSPECIFIED., .F., .F.,
 ( 4, 1, 1, 1, 1, 1, 1, 1, 1, 1, 1, 1, 1, 1, 1, 1, 4 ),
 ( 0.000000000000000000, 0.06250000000000000000, 0.1250000000000000000, 0.1875000000000000000, 0.2500000000000000000, 0.3125000000000000000, 0.3750000000000000000, 0.4375000000000000000, 0.5000000000000000000, 0.5625000000000000000, 0.6250000000000000000, 0.6875000000000000000, 0.7500000000000000000, 0.8125000000000000000, 0.8750000000000000000, 0.9375000000000000000, 0.9999968116805088014 ),
 .UNSPECIFIED. ) ;
#17733=ORIENTED_EDGE ( 'NONE', *, *, #4511, .T. ) ;
#17745=ORIENTED_EDGE ( 'NONE', *, *, #5815, .T. ) ;
#17789=VERTEX_POINT ( 'NONE', #22468 ) ;
#17843=ORIENTED_EDGE ( 'NONE', *, *, #21897, .F. ) ;
#17917=VERTEX_POINT ( 'NONE', #1611 ) ;
#17936=CARTESIAN_POINT ( 'NONE',  ( 12.97541421502999981, -3662.340907203999905, 2257.594921553999939 ) ) ;
#18059=CARTESIAN_POINT ( 'NONE',  ( 15.33658054938999982, -3660.585448001000259, 2257.909769185999721 ) ) ;
#18179=DIRECTION ( 'NONE',  ( 1.000000000000000000, 0.000000000000000000, 0.000000000000000000 ) ) ;
#18374=DIRECTION ( 'NONE',  ( 0.000000000000000000, 0.000000000000000000, 1.000000000000000000 ) ) ;
#18381=EDGE_LOOP ( 'NONE', ( #13333, #2179, #21, #17733, #11003, #19413, #14965, #24 ) ) ;
#18414=CARTESIAN_POINT ( 'NONE',  ( 9.855200508393229697, -3659.504999998446692, 2257.962940200992307 ) ) ;
#18421=VECTOR ( 'NONE', #7245, 1000.000000000000000 ) ;
#18576=DIRECTION ( 'NONE',  ( 0.000000000000000000, -1.000000000000000000, 0.000000000000000000 ) ) ;
#18609=CARTESIAN_POINT ( 'NONE',  ( 12.69999999999999929, -3659.504999999999654, 2272.030000000000200 ) ) ;
#18631=ORIENTED_EDGE ( 'NONE', *, *, #14152, .F. ) ;
#18644=PLANE ( 'NONE',  #2547 ) ;
#18765=DIRECTION ( 'NONE',  ( 1.000000000000000000, 0.000000000000000000, 0.000000000000000000 ) ) ;
#18844=CARTESIAN_POINT ( 'NONE',  ( 13.24918551347000140, -3656.709137200999521, 2257.605105471000115 ) ) ;
#18912=DIRECTION ( 'NONE',  ( 0.000000000000000000, 1.000000000000000000, 0.000000000000000000 ) ) ;
#18929=FACE_OUTER_BOUND ( 'NONE', #17499, .T. ) ;
#19136=VECTOR ( 'NONE', #18912, 1000.000000000000000 ) ;
#19203=CARTESIAN_POINT ( 'NONE',  ( 15.21772229205999949, -3658.170722075999947, 2257.881333375999930 ) ) ;
#19413=ORIENTED_EDGE ( 'NONE', *, *, #10239, .T. ) ;
#19430=CARTESIAN_POINT ( 'NONE',  ( 10.06337286646999907, -3658.424665316000301, 2257.909780569999839 ) ) ;
#19431=CARTESIAN_POINT ( 'NONE',  ( 10.68478392833999990, -3661.519597158000124, 2257.776259854999807 ) ) ;
#19457=CARTESIAN_POINT ( 'NONE',  ( 12.69999999999999929, -3648.710000000000036, 2268.705139999999574 ) ) ;
#19497=ORIENTED_EDGE ( 'NONE', *, *, #531, .T. ) ;
#19544=CARTESIAN_POINT ( 'NONE',  ( 10.68485228337000059, -3657.490333022999948, 2257.776247070999943 ) ) ;
#19545=DIRECTION ( 'NONE',  ( 0.000000000000000000, 0.000000000000000000, -1.000000000000000000 ) ) ;
#19565=VERTEX_POINT ( 'NONE', #16293 ) ;
#19713=CARTESIAN_POINT ( 'NONE',  ( 15.53591867179932073, -3659.780168290938946, 2257.960586820520803 ) ) ;
#19785=CARTESIAN_POINT ( 'NONE',  ( 10.89511648704999836, -3657.299999577000108, 2257.739442794000297 ) ) ;
#19824=CARTESIAN_POINT ( 'NONE',  ( 13.78126912685999983, -3662.141243252000095, 2257.644351290000031 ) ) ;
#19825=CARTESIAN_POINT ( 'NONE',  ( 12.70000000000000107, -3649.471999999999753, 2275.817139999999654 ) ) ;
#20019=CARTESIAN_POINT ( 'NONE',  ( 15.54479999999999862, -3659.504999999999654, 2272.030000000000200 ) ) ;
#20077=DIRECTION ( 'NONE',  ( 0.000000000000000000, 1.000000000000000000, 0.000000000000000000 ) ) ;
#20108=ADVANCED_FACE ( 'NONE', ( #1121 ), #4338, .T. ) ;
#20304=CARTESIAN_POINT ( 'NONE',  ( 15.54479999999999862, -3659.504999999999654, 2272.030000000000200 ) ) ;
#20332=ORIENTED_EDGE ( 'NONE', *, *, #15553, .F. ) ;
#20423=DIRECTION ( 'NONE',  ( 0.000000000000000000, 0.000000000000000000, 1.000000000000000000 ) ) ;
#20441=PRODUCT_DEFINITION_SHAPE ( 'NONE', 'NONE',  #22928 ) ;
#20459=DIRECTION ( 'NONE',  ( 0.000000000000000000, 0.000000000000000000, -1.000000000000000000 ) ) ;
#20479=CARTESIAN_POINT ( 'NONE',  ( 12.69999999999999929, -3649.471999999999753, 2268.705139999999574 ) ) ;
#20484=CYLINDRICAL_SURFACE ( 'NONE', #13930, 2.844799999999999773 ) ;
#20695=DIRECTION ( 'NONE',  ( 0.000000000000000000, -1.000000000000000000, 0.000000000000000000 ) ) ;
#20971=AXIS2_PLACEMENT_3D ( 'NONE', #3651, #12446, #18179 ) ;
#21007=SHAPE_REPRESENTATION_RELATIONSHIP ( 'NONE' , 'NONE' ,  #6985, #15234 ) ;
#21045=AXIS2_PLACEMENT_3D ( 'NONE', #10631, #13690, #22580 ) ;
#21072=VECTOR ( 'NONE', #20077, 1000.000000000000000 ) ;
#21077=CARTESIAN_POINT ( 'NONE',  ( 12.97550722921000066, -3656.669101291999596, 2257.594923726999696 ) ) ;
#21094=CIRCLE ( 'NONE', #15469, 6.349999999999855760 ) ;
#21103=DIRECTION ( 'NONE',  ( 0.000000000000000000, 0.000000000000000000, -1.000000000000000000 ) ) ;
#21126=( LENGTH_UNIT ( ) NAMED_UNIT ( * ) SI_UNIT ( .MILLI., .METRE. ) );
#21221=DIRECTION ( 'NONE',  ( 0.000000000000000000, -1.000000000000000000, 0.000000000000000000 ) ) ;
#21267=DIRECTION ( 'NONE',  ( 0.000000000000000000, -1.000000000000000000, 0.000000000000000000 ) ) ;
#21423=CARTESIAN_POINT ( 'NONE',  ( 12.69999999999999929, -3656.660200000000259, 2257.592639999999847 ) ) ;
#21540=EDGE_CURVE ( 'NONE', #7425, #5186, #3206, .T. ) ;
#21542=CARTESIAN_POINT ( 'NONE',  ( 11.88149704131999940, -3656.775771668999823, 2257.621751704000417 ) ) ;
#21559=ORIENTED_EDGE ( 'NONE', *, *, #1366, .T. ) ;
#21597=DIRECTION ( 'NONE',  ( 0.000000000000000000, 0.000000000000000000, 1.000000000000000000 ) ) ;
#21639=CARTESIAN_POINT ( 'NONE',  ( 15.54479972192533488, -3659.504999998566745, 2257.962943247991007 ) ) ;
#21897=EDGE_CURVE ( 'NONE', #7027, #19565, #16689, .T. ) ;
#21921=CARTESIAN_POINT ( 'NONE',  ( 12.70000000000000107, -3648.710000000000036, 2279.817639999999756 ) ) ;
#22030=APPLICATION_CONTEXT ( 'configuration controlled 3d designs of mechanical parts and assemblies' ) ;
#22131=CIRCLE ( 'NONE', #10550, 0.7619999999999294005 ) ;
#22203=CARTESIAN_POINT ( 'NONE',  ( 9.855200508393229697, -3659.504999998446692, 2257.962940200992307 ) ) ;
#22205=CYLINDRICAL_SURFACE ( 'NONE', #3450, 2.844799999999999773 ) ;
#22217=CYLINDRICAL_SURFACE ( 'NONE', #14437, 11.11249999999985860 ) ;
#22245=ORIENTED_EDGE ( 'NONE', *, *, #21897, .T. ) ;
#22263=CARTESIAN_POINT ( 'NONE',  ( 12.69999999999999929, -3655.060000000000400, 2275.055139999999483 ) ) ;
#22288=CARTESIAN_POINT ( 'NONE',  ( 12.69999999999999929, -3648.710000000000036, 2268.705139999999574 ) ) ;
#22402=DIRECTION ( 'NONE',  ( 1.000000000000000000, 0.000000000000000000, 3.996303350731721563E-14 ) ) ;
#22466=B_SPLINE_CURVE_WITH_KNOTS ( 'NONE', 3,
 ( #2910, #3258, #6676, #10049, #10285, #13925, #5144, #4898, #17196, #19431, #17428, #1490, #13577, #8305, #17312, #15449, #1382, #14043, #1258 ),
 .UNSPECIFIED., .F., .F.,
 ( 4, 1, 1, 1, 1, 1, 1, 1, 1, 1, 1, 1, 1, 1, 1, 1, 4 ),
 ( 3.168591426078622932E-06, 0.06250000000000000000, 0.1250000000000000000, 0.1875000000000000000, 0.2500000000000000000, 0.3125000000000000000, 0.3750000000000000000, 0.4375000000000000000, 0.5000000000000000000, 0.5625000000000000000, 0.6250000000000000000, 0.6875000000000000000, 0.7500000000000000000, 0.8125000000000000000, 0.8750000000000000000, 0.9375000000000000000, 1.000000000000000000 ),
 .UNSPECIFIED. ) ;
#22468=CARTESIAN_POINT ( 'NONE',  ( 15.54479972196000048, -3659.504985917999875, 2257.962943248000101 ) ) ;
#22511=DIRECTION ( 'NONE',  ( 0.000000000000000000, 0.000000000000000000, -1.000000000000000000 ) ) ;
#22580=DIRECTION ( 'NONE',  ( 1.000000000000000000, 0.000000000000000000, 3.996303350731721563E-14 ) ) ;
#22584=CARTESIAN_POINT ( 'NONE',  ( 13.78135004281000064, -3656.868789907000064, 2257.644359223000265 ) ) ;
#22896=CARTESIAN_POINT ( 'NONE',  ( 12.69999999999999929, -3649.471999999999753, 2268.705139999999574 ) ) ;
#22901=CARTESIAN_POINT ( 'NONE',  ( 9.855199999999999960, -3659.504999999999654, 2272.030000000000200 ) ) ;
#22925=CARTESIAN_POINT ( 'NONE',  ( 10.18227723364999981, -3658.170723028000339, 2257.881333495000035 ) ) ;
#22928=PRODUCT_DEFINITION ( 'UNKNOWN', '', #8248, #1275 ) ;
#23094=( NAMED_UNIT ( * ) SI_UNIT ( $, .STERADIAN. ) SOLID_ANGLE_UNIT ( ) );
#23117=ORIENTED_EDGE ( 'NONE', *, *, #15951, .T. ) ;
#23194=COLOUR_RGB('Sky Blue',0.24,0.69,0.87);
#23195=FILL_AREA_STYLE_COLOUR('',#23194);
#23196=FILL_AREA_STYLE('',(#23195));
#23197=SURFACE_STYLE_FILL_AREA(#23196);
#23198=SURFACE_SIDE_STYLE('',(#23197));
#23199=SURFACE_STYLE_USAGE(.BOTH.,#23198);
#23200=PRESENTATION_STYLE_ASSIGNMENT((#23199));
#23236=STYLED_ITEM('',(#23200),#5838);
#23237=MECHANICAL_DESIGN_GEOMETRIC_PRESENTATION_REPRESENTATION('',(#23236),#2257);
ENDSEC;
END-ISO-10303-21;
